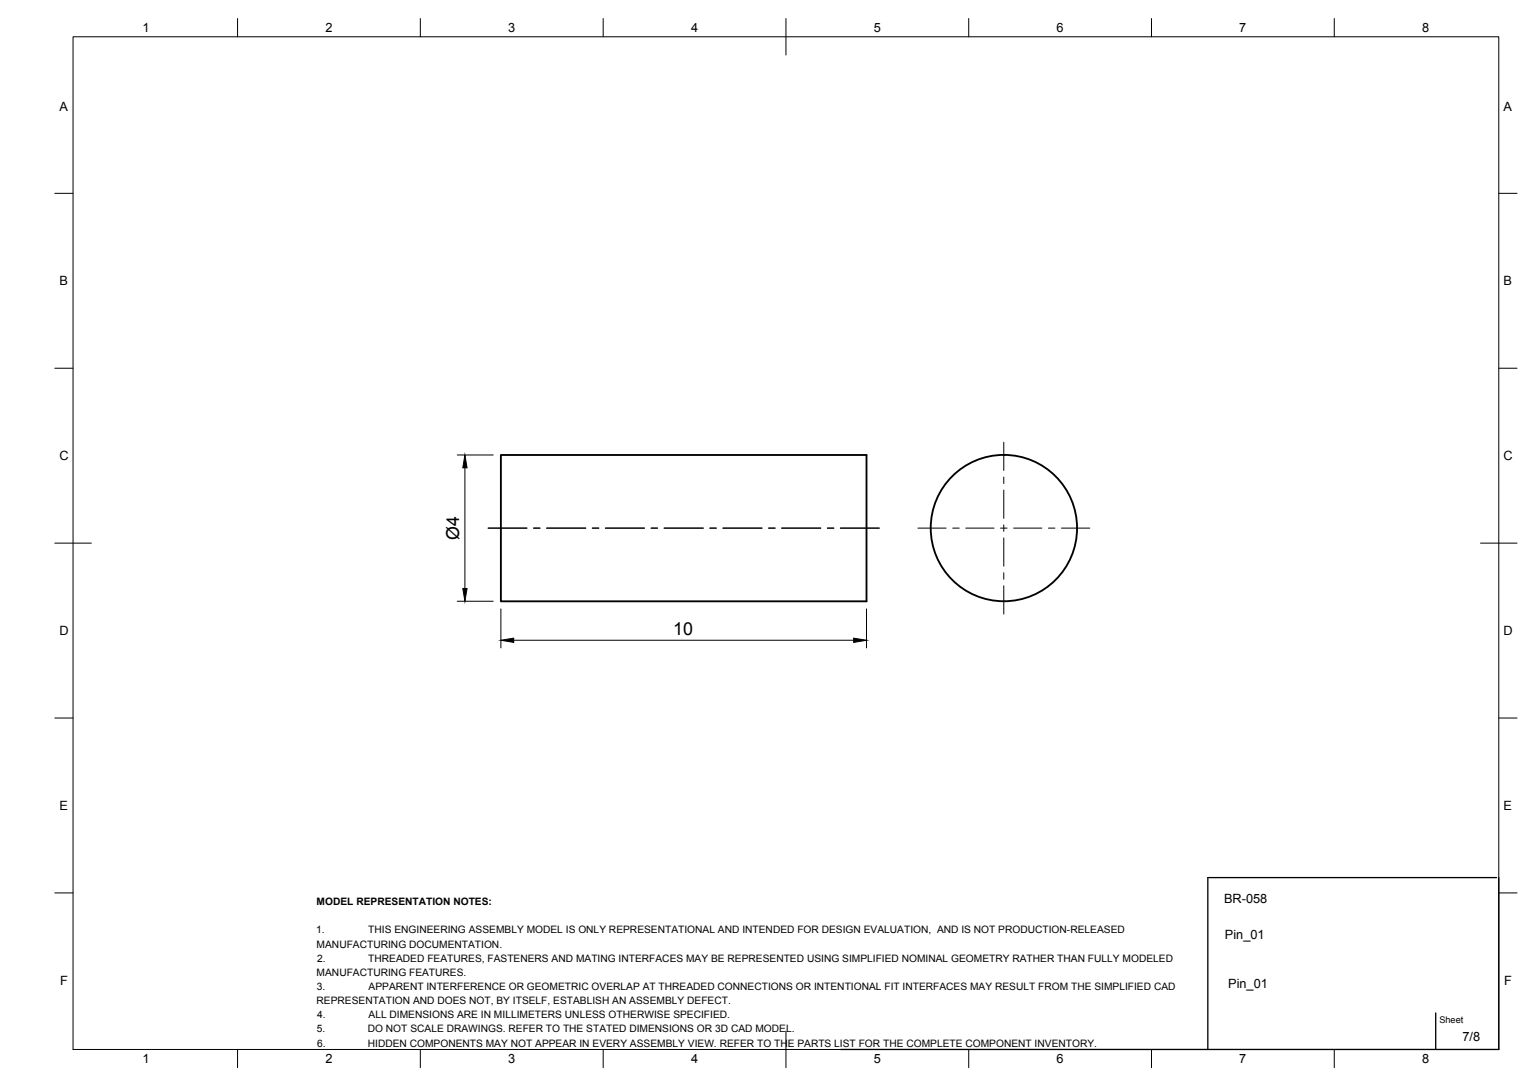
ISO-10303-21;
HEADER;
/* Generated by software containing ST-Developer
 * from STEP Tools, Inc. (www.steptools.com) 
 */

FILE_DESCRIPTION(
/* description */ (''),
/* implementation_level */ '2;1');

FILE_NAME(
/* name */ 'Pin_01.step',
/* time_stamp */ '2026-10-12T16:07:47-07:00',
/* author */ (''),
/* organization */ (''),
/* preprocessor_version */ 'ST-DEVELOPER v20.2',
/* originating_system */ 'Autodesk Translation Framework v15.15.0.0',
/* authorisation */ '');

FILE_SCHEMA (('AUTOMOTIVE_DESIGN { 1 0 10303 214 3 1 1 }'));
ENDSEC;

DATA;
#10=MECHANICAL_DESIGN_GEOMETRIC_PRESENTATION_REPRESENTATION('',(#97),#8779);
#83=SHAPE_REPRESENTATION_RELATIONSHIP('SRR','None',#8812,#90);
#90=ADVANCED_BREP_SHAPE_REPRESENTATION('',(#107),#8775);
#97=STYLED_ITEM('',(#8854),#107);
#107=MANIFOLD_SOLID_BREP('Body1',#5117);
#301=CIRCLE('',#5542,2.00038918348039);
#302=CIRCLE('',#5543,2.00038918348039);
#462=CYLINDRICAL_SURFACE('',#5541,2.00038918348039);
#677=FACE_OUTER_BOUND('',#990,.T.);
#678=FACE_OUTER_BOUND('',#991,.T.);
#679=FACE_OUTER_BOUND('',#992,.T.);
#990=EDGE_LOOP('',(#4416,#4417,#4418,#4419));
#991=EDGE_LOOP('',(#4420));
#992=EDGE_LOOP('',(#4421));
#1540=LINE('',#8438,#2025);
#2025=VECTOR('',#6860,2.00038918348039);
#2446=VERTEX_POINT('',#8435);
#2447=VERTEX_POINT('',#8437);
#3112=EDGE_CURVE('',#2446,#2446,#301,.T.);
#3113=EDGE_CURVE('',#2446,#2447,#1540,.T.);
#3114=EDGE_CURVE('',#2447,#2447,#302,.T.);
#4416=ORIENTED_EDGE('',*,*,#3112,.T.);
#4417=ORIENTED_EDGE('',*,*,#3113,.T.);
#4418=ORIENTED_EDGE('',*,*,#3114,.F.);
#4419=ORIENTED_EDGE('',*,*,#3113,.F.);
#4420=ORIENTED_EDGE('',*,*,#3114,.T.);
#4421=ORIENTED_EDGE('',*,*,#3112,.F.);
#4808=PLANE('',#5544);
#4809=PLANE('',#5545);
#5039=ADVANCED_FACE('',(#677),#462,.T.);
#5040=ADVANCED_FACE('',(#678),#4808,.F.);
#5041=ADVANCED_FACE('',(#679),#4809,.T.);
#5117=CLOSED_SHELL('',(#5039,#5040,#5041));
#5540=AXIS2_PLACEMENT_3D('',#8433,#6854,#6855);
#5541=AXIS2_PLACEMENT_3D('',#8434,#6856,#6857);
#5542=AXIS2_PLACEMENT_3D('',#8436,#6858,#6859);
#5543=AXIS2_PLACEMENT_3D('',#8439,#6861,#6862);
#5544=AXIS2_PLACEMENT_3D('',#8440,#6863,#6864);
#5545=AXIS2_PLACEMENT_3D('',#8441,#6865,#6866);
#6854=DIRECTION('axis',(0.,0.,1.));
#6855=DIRECTION('refdir',(1.,0.,0.));
#6856=DIRECTION('center_axis',(0.,1.,0.));
#6857=DIRECTION('ref_axis',(1.,0.,0.));
#6858=DIRECTION('center_axis',(0.,-1.,0.));
#6859=DIRECTION('ref_axis',(1.,0.,0.));
#6860=DIRECTION('',(0.,-1.,0.));
#6861=DIRECTION('center_axis',(0.,-1.,0.));
#6862=DIRECTION('ref_axis',(1.,0.,0.));
#6863=DIRECTION('center_axis',(0.,1.,0.));
#6864=DIRECTION('ref_axis',(1.,0.,0.));
#6865=DIRECTION('center_axis',(0.,1.,0.));
#6866=DIRECTION('ref_axis',(0.,0.,1.));
#8433=CARTESIAN_POINT('',(0.,0.,0.));
#8434=CARTESIAN_POINT('Origin',(0.,0.,92.461739559435));
#8435=CARTESIAN_POINT('',(-2.00038918348039,4.,92.461739559435));
#8436=CARTESIAN_POINT('Origin',(0.,4.,92.461739559435));
#8437=CARTESIAN_POINT('',(-2.00038918348039,-6.,92.461739559435));
#8438=CARTESIAN_POINT('',(-2.00038918348039,0.,92.461739559435));
#8439=CARTESIAN_POINT('Origin',(0.,-6.,92.461739559435));
#8440=CARTESIAN_POINT('Origin',(0.,-6.,92.461739559435));
#8441=CARTESIAN_POINT('Origin',(1.,4.,47.9085167784579));
#8766=UNCERTAINTY_MEASURE_WITH_UNIT(LENGTH_MEASURE(0.01),#8780,
'DISTANCE_ACCURACY_VALUE',
'Maximum model space distance between geometric entities at asserted c
onnectivities');
#8770=UNCERTAINTY_MEASURE_WITH_UNIT(LENGTH_MEASURE(0.01),#8780,
'DISTANCE_ACCURACY_VALUE',
'Maximum model space distance between geometric entities at asserted c
onnectivities');
#8775=(
GEOMETRIC_REPRESENTATION_CONTEXT(3)
GLOBAL_UNCERTAINTY_ASSIGNED_CONTEXT((#8766))
GLOBAL_UNIT_ASSIGNED_CONTEXT((#8780,#8782,#8783))
REPRESENTATION_CONTEXT('','3D')
);
#8779=(
GEOMETRIC_REPRESENTATION_CONTEXT(3)
GLOBAL_UNCERTAINTY_ASSIGNED_CONTEXT((#8770))
GLOBAL_UNIT_ASSIGNED_CONTEXT((#8780,#8782,#8783))
REPRESENTATION_CONTEXT('','3D')
);
#8780=(
LENGTH_UNIT()
NAMED_UNIT(*)
SI_UNIT(.MILLI.,.METRE.)
);
#8782=(
NAMED_UNIT(*)
PLANE_ANGLE_UNIT()
SI_UNIT($,.RADIAN.)
);
#8783=(
NAMED_UNIT(*)
SI_UNIT($,.STERADIAN.)
SOLID_ANGLE_UNIT()
);
#8788=SHAPE_DEFINITION_REPRESENTATION(#8796,#8812);
#8796=PRODUCT_DEFINITION_SHAPE('',$,#8821);
#8812=SHAPE_REPRESENTATION('',(#5540),#8775);
#8816=PRODUCT_DEFINITION_CONTEXT('part definition',#8842,'design');
#8821=PRODUCT_DEFINITION('Pin_01','Pin_01',#8829,#8816);
#8829=PRODUCT_DEFINITION_FORMATION('',$,#8848);
#8842=APPLICATION_CONTEXT(
'Core Data for Automotive Mechanical Design Process');
#8843=PRODUCT_CONTEXT('part definition',#8842,'mechanical');
#8848=PRODUCT('Pin_01','Pin_01',$,(#8843));
#8854=PRESENTATION_STYLE_ASSIGNMENT((#8859));
#8859=SURFACE_STYLE_USAGE(.BOTH.,#8864);
#8864=SURFACE_SIDE_STYLE('',(#8869));
#8869=SURFACE_STYLE_FILL_AREA(#8874);
#8874=FILL_AREA_STYLE('Opaque(85,170,0)',(#8879));
#8879=FILL_AREA_STYLE_COLOUR('Opaque(85,170,0)',#8884);
#8884=COLOUR_RGB('Opaque(85,170,0)', 0.66274510, 0.83137255, 0.94901961);
ENDSEC;
END-ISO-10303-21;
